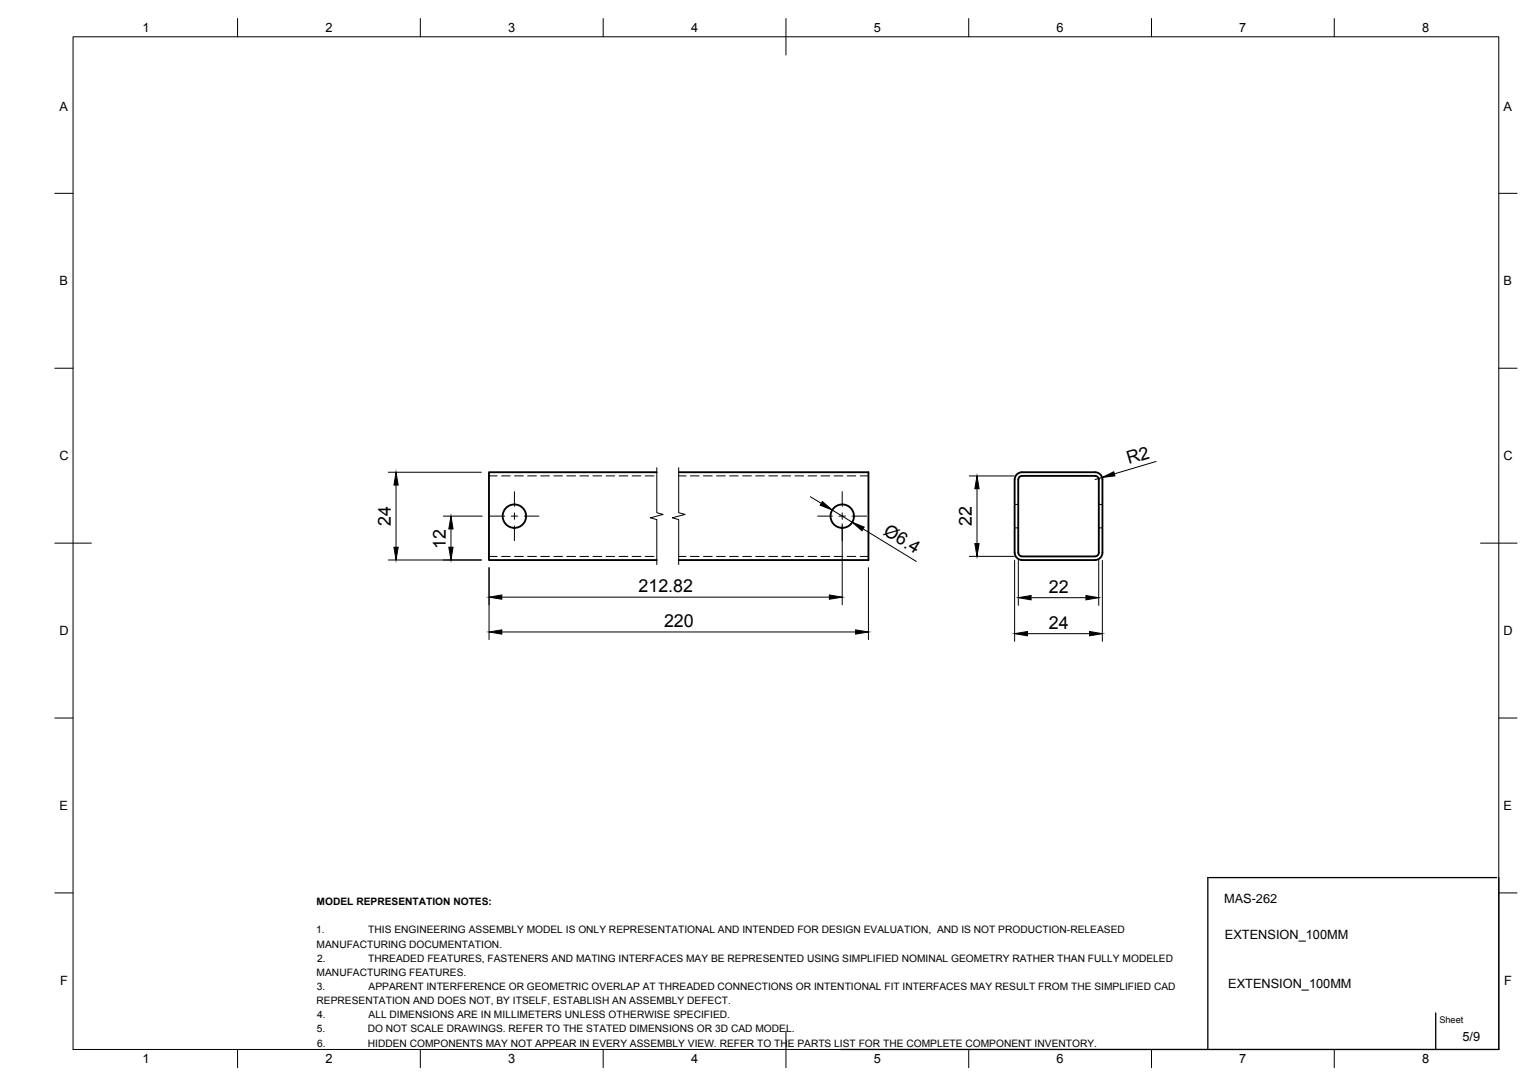
ISO-10303-21;
HEADER;
/* Generated by software containing ST-Developer
 * from STEP Tools, Inc. (www.steptools.com) 
 */

FILE_DESCRIPTION(
/* description */ (''),
/* implementation_level */ '2;1');

FILE_NAME(
/* name */ 'EXTENSION_100MM.step',
/* time_stamp */ '2026-10-07T02:13:48+06:00',
/* author */ (''),
/* organization */ (''),
/* preprocessor_version */ 'ST-DEVELOPER v20.2',
/* originating_system */ 'Autodesk Translation Framework v15.15.0.0',
/* authorisation */ '');

FILE_SCHEMA (('AUTOMOTIVE_DESIGN { 1 0 10303 214 3 1 1 }'));
ENDSEC;

DATA;
#10=MECHANICAL_DESIGN_GEOMETRIC_PRESENTATION_REPRESENTATION('',(#116),#17042);
#92=SHAPE_REPRESENTATION_RELATIONSHIP('SRR','None',#17088,#104);
#104=ADVANCED_BREP_SHAPE_REPRESENTATION('',(#128),#17032);
#116=STYLED_ITEM('',(#17154),#128);
#128=MANIFOLD_SOLID_BREP('Body1',#8117);
#148=FACE_BOUND('',#1141,.T.);
#149=FACE_BOUND('',#1145,.T.);
#150=FACE_BOUND('',#1146,.T.);
#151=FACE_BOUND('',#1151,.T.);
#152=FACE_BOUND('',#1152,.T.);
#153=FACE_BOUND('',#1157,.T.);
#154=FACE_BOUND('',#1158,.T.);
#155=FACE_BOUND('',#1163,.T.);
#156=FACE_BOUND('',#1164,.T.);
#157=FACE_BOUND('',#1167,.T.);
#360=PLANE('',#8614);
#361=PLANE('',#8623);
#362=PLANE('',#8626);
#363=PLANE('',#8629);
#364=PLANE('',#8632);
#365=PLANE('',#8635);
#366=PLANE('',#8638);
#367=PLANE('',#8641);
#368=PLANE('',#8644);
#369=PLANE('',#8647);
#649=FACE_OUTER_BOUND('',#1136,.T.);
#650=FACE_OUTER_BOUND('',#1137,.T.);
#651=FACE_OUTER_BOUND('',#1138,.T.);
#652=FACE_OUTER_BOUND('',#1139,.T.);
#653=FACE_OUTER_BOUND('',#1140,.T.);
#654=FACE_OUTER_BOUND('',#1142,.T.);
#655=FACE_OUTER_BOUND('',#1143,.T.);
#656=FACE_OUTER_BOUND('',#1144,.T.);
#657=FACE_OUTER_BOUND('',#1147,.T.);
#658=FACE_OUTER_BOUND('',#1148,.T.);
#659=FACE_OUTER_BOUND('',#1149,.T.);
#660=FACE_OUTER_BOUND('',#1150,.T.);
#661=FACE_OUTER_BOUND('',#1153,.T.);
#662=FACE_OUTER_BOUND('',#1154,.T.);
#663=FACE_OUTER_BOUND('',#1155,.T.);
#664=FACE_OUTER_BOUND('',#1156,.T.);
#665=FACE_OUTER_BOUND('',#1159,.T.);
#666=FACE_OUTER_BOUND('',#1160,.T.);
#667=FACE_OUTER_BOUND('',#1161,.T.);
#668=FACE_OUTER_BOUND('',#1162,.T.);
#669=FACE_OUTER_BOUND('',#1165,.T.);
#670=FACE_OUTER_BOUND('',#1166,.T.);
#1136=EDGE_LOOP('',(#6001,#6002,#6003,#6004));
#1137=EDGE_LOOP('',(#6005,#6006,#6007,#6008));
#1138=EDGE_LOOP('',(#6009,#6010,#6011,#6012));
#1139=EDGE_LOOP('',(#6013,#6014,#6015,#6016));
#1140=EDGE_LOOP('',(#6017,#6018,#6019,#6020,#6021,#6022,#6023,#6024));
#1141=EDGE_LOOP('',(#6025,#6026,#6027,#6028,#6029,#6030,#6031,#6032));
#1142=EDGE_LOOP('',(#6033,#6034,#6035,#6036));
#1143=EDGE_LOOP('',(#6037,#6038,#6039,#6040));
#1144=EDGE_LOOP('',(#6041,#6042,#6043,#6044));
#1145=EDGE_LOOP('',(#6045));
#1146=EDGE_LOOP('',(#6046));
#1147=EDGE_LOOP('',(#6047,#6048,#6049,#6050));
#1148=EDGE_LOOP('',(#6051,#6052,#6053,#6054));
#1149=EDGE_LOOP('',(#6055,#6056,#6057,#6058));
#1150=EDGE_LOOP('',(#6059,#6060,#6061,#6062));
#1151=EDGE_LOOP('',(#6063));
#1152=EDGE_LOOP('',(#6064));
#1153=EDGE_LOOP('',(#6065,#6066,#6067,#6068));
#1154=EDGE_LOOP('',(#6069,#6070,#6071,#6072));
#1155=EDGE_LOOP('',(#6073,#6074,#6075,#6076));
#1156=EDGE_LOOP('',(#6077,#6078,#6079,#6080));
#1157=EDGE_LOOP('',(#6081));
#1158=EDGE_LOOP('',(#6082));
#1159=EDGE_LOOP('',(#6083,#6084,#6085,#6086));
#1160=EDGE_LOOP('',(#6087,#6088,#6089,#6090));
#1161=EDGE_LOOP('',(#6091,#6092,#6093,#6094));
#1162=EDGE_LOOP('',(#6095,#6096,#6097,#6098));
#1163=EDGE_LOOP('',(#6099));
#1164=EDGE_LOOP('',(#6100));
#1165=EDGE_LOOP('',(#6101,#6102,#6103,#6104));
#1166=EDGE_LOOP('',(#6105,#6106,#6107,#6108,#6109,#6110,#6111,#6112));
#1167=EDGE_LOOP('',(#6113,#6114,#6115,#6116,#6117,#6118,#6119,#6120));
#1642=CIRCLE('',#8603,3.20000000000001);
#1643=CIRCLE('',#8604,3.20000000000001);
#1644=CIRCLE('',#8606,3.20000000000001);
#1645=CIRCLE('',#8607,3.20000000000001);
#1646=CIRCLE('',#8609,3.2);
#1647=CIRCLE('',#8610,3.2);
#1648=CIRCLE('',#8612,3.2);
#1649=CIRCLE('',#8613,3.2);
#1650=CIRCLE('',#8615,2.);
#1651=CIRCLE('',#8616,2.);
#1652=CIRCLE('',#8617,2.);
#1653=CIRCLE('',#8618,2.);
#1654=CIRCLE('',#8619,0.999999999999999);
#1655=CIRCLE('',#8620,0.999999999999999);
#1656=CIRCLE('',#8621,0.999999999999999);
#1657=CIRCLE('',#8622,1.);
#1658=CIRCLE('',#8625,0.999999999999999);
#1659=CIRCLE('',#8628,0.999999999999999);
#1660=CIRCLE('',#8631,1.);
#1661=CIRCLE('',#8634,0.999999999999999);
#1662=CIRCLE('',#8637,2.);
#1663=CIRCLE('',#8640,2.);
#1664=CIRCLE('',#8643,2.);
#1665=CIRCLE('',#8646,2.);
#2301=LINE('',#12839,#2879);
#2302=LINE('',#12845,#2880);
#2303=LINE('',#12851,#2881);
#2304=LINE('',#12857,#2882);
#2305=LINE('',#12864,#2883);
#2306=LINE('',#12868,#2884);
#2307=LINE('',#12872,#2885);
#2308=LINE('',#12875,#2886);
#2309=LINE('',#12880,#2887);
#2310=LINE('',#12884,#2888);
#2311=LINE('',#12888,#2889);
#2312=LINE('',#12891,#2890);
#2313=LINE('',#12894,#2891);
#2314=LINE('',#12896,#2892);
#2315=LINE('',#12897,#2893);
#2316=LINE('',#12901,#2894);
#2317=LINE('',#12904,#2895);
#2318=LINE('',#12905,#2896);
#2319=LINE('',#12909,#2897);
#2320=LINE('',#12912,#2898);
#2321=LINE('',#12913,#2899);
#2322=LINE('',#12917,#2900);
#2323=LINE('',#12920,#2901);
#2324=LINE('',#12921,#2902);
#2325=LINE('',#12926,#2903);
#2326=LINE('',#12928,#2904);
#2327=LINE('',#12929,#2905);
#2328=LINE('',#12933,#2906);
#2329=LINE('',#12936,#2907);
#2330=LINE('',#12937,#2908);
#2331=LINE('',#12941,#2909);
#2332=LINE('',#12944,#2910);
#2333=LINE('',#12945,#2911);
#2334=LINE('',#12949,#2912);
#2335=LINE('',#12952,#2913);
#2336=LINE('',#12953,#2914);
#2879=VECTOR('',#10218,3.20000000000001);
#2880=VECTOR('',#10225,3.20000000000001);
#2881=VECTOR('',#10232,3.2);
#2882=VECTOR('',#10239,3.2);
#2883=VECTOR('',#10246,20.);
#2884=VECTOR('',#10249,20.);
#2885=VECTOR('',#10252,20.);
#2886=VECTOR('',#10255,20.);
#2887=VECTOR('',#10258,20.);
#2888=VECTOR('',#10261,20.);
#2889=VECTOR('',#10264,20.);
#2890=VECTOR('',#10267,20.);
#2891=VECTOR('',#10270,20.);
#2892=VECTOR('',#10271,20.);
#2893=VECTOR('',#10272,20.);
#2894=VECTOR('',#10277,20.);
#2895=VECTOR('',#10280,20.);
#2896=VECTOR('',#10281,20.);
#2897=VECTOR('',#10286,20.);
#2898=VECTOR('',#10289,20.);
#2899=VECTOR('',#10290,20.);
#2900=VECTOR('',#10295,20.);
#2901=VECTOR('',#10298,20.);
#2902=VECTOR('',#10299,20.);
#2903=VECTOR('',#10306,20.);
#2904=VECTOR('',#10307,20.);
#2905=VECTOR('',#10308,20.);
#2906=VECTOR('',#10313,20.);
#2907=VECTOR('',#10316,20.);
#2908=VECTOR('',#10317,20.);
#2909=VECTOR('',#10322,20.);
#2910=VECTOR('',#10325,20.);
#2911=VECTOR('',#10326,20.);
#2912=VECTOR('',#10331,20.);
#2913=VECTOR('',#10334,20.);
#2914=VECTOR('',#10335,20.);
#3465=VERTEX_POINT('',#12836);
#3466=VERTEX_POINT('',#12838);
#3467=VERTEX_POINT('',#12842);
#3468=VERTEX_POINT('',#12844);
#3469=VERTEX_POINT('',#12848);
#3470=VERTEX_POINT('',#12850);
#3471=VERTEX_POINT('',#12854);
#3472=VERTEX_POINT('',#12856);
#3473=VERTEX_POINT('',#12860);
#3474=VERTEX_POINT('',#12861);
#3475=VERTEX_POINT('',#12863);
#3476=VERTEX_POINT('',#12865);
#3477=VERTEX_POINT('',#12867);
#3478=VERTEX_POINT('',#12869);
#3479=VERTEX_POINT('',#12871);
#3480=VERTEX_POINT('',#12873);
#3481=VERTEX_POINT('',#12876);
#3482=VERTEX_POINT('',#12877);
#3483=VERTEX_POINT('',#12879);
#3484=VERTEX_POINT('',#12881);
#3485=VERTEX_POINT('',#12883);
#3486=VERTEX_POINT('',#12885);
#3487=VERTEX_POINT('',#12887);
#3488=VERTEX_POINT('',#12889);
#3489=VERTEX_POINT('',#12893);
#3490=VERTEX_POINT('',#12895);
#3491=VERTEX_POINT('',#12899);
#3492=VERTEX_POINT('',#12903);
#3493=VERTEX_POINT('',#12907);
#3494=VERTEX_POINT('',#12911);
#3495=VERTEX_POINT('',#12915);
#3496=VERTEX_POINT('',#12919);
#3497=VERTEX_POINT('',#12925);
#3498=VERTEX_POINT('',#12927);
#3499=VERTEX_POINT('',#12931);
#3500=VERTEX_POINT('',#12935);
#3501=VERTEX_POINT('',#12939);
#3502=VERTEX_POINT('',#12943);
#3503=VERTEX_POINT('',#12947);
#3504=VERTEX_POINT('',#12951);
#4368=EDGE_CURVE('',#3465,#3465,#1642,.T.);
#4369=EDGE_CURVE('',#3465,#3466,#2301,.T.);
#4370=EDGE_CURVE('',#3466,#3466,#1643,.T.);
#4371=EDGE_CURVE('',#3467,#3467,#1644,.T.);
#4372=EDGE_CURVE('',#3467,#3468,#2302,.T.);
#4373=EDGE_CURVE('',#3468,#3468,#1645,.T.);
#4374=EDGE_CURVE('',#3469,#3469,#1646,.T.);
#4375=EDGE_CURVE('',#3469,#3470,#2303,.T.);
#4376=EDGE_CURVE('',#3470,#3470,#1647,.T.);
#4377=EDGE_CURVE('',#3471,#3471,#1648,.T.);
#4378=EDGE_CURVE('',#3471,#3472,#2304,.T.);
#4379=EDGE_CURVE('',#3472,#3472,#1649,.T.);
#4380=EDGE_CURVE('',#3473,#3474,#1650,.T.);
#4381=EDGE_CURVE('',#3474,#3475,#2305,.T.);
#4382=EDGE_CURVE('',#3475,#3476,#1651,.T.);
#4383=EDGE_CURVE('',#3476,#3477,#2306,.T.);
#4384=EDGE_CURVE('',#3477,#3478,#1652,.T.);
#4385=EDGE_CURVE('',#3478,#3479,#2307,.T.);
#4386=EDGE_CURVE('',#3479,#3480,#1653,.T.);
#4387=EDGE_CURVE('',#3480,#3473,#2308,.T.);
#4388=EDGE_CURVE('',#3481,#3482,#1654,.T.);
#4389=EDGE_CURVE('',#3482,#3483,#2309,.T.);
#4390=EDGE_CURVE('',#3483,#3484,#1655,.T.);
#4391=EDGE_CURVE('',#3484,#3485,#2310,.T.);
#4392=EDGE_CURVE('',#3485,#3486,#1656,.T.);
#4393=EDGE_CURVE('',#3486,#3487,#2311,.T.);
#4394=EDGE_CURVE('',#3487,#3488,#1657,.T.);
#4395=EDGE_CURVE('',#3488,#3481,#2312,.T.);
#4396=EDGE_CURVE('',#3489,#3482,#2313,.T.);
#4397=EDGE_CURVE('',#3490,#3489,#2314,.T.);
#4398=EDGE_CURVE('',#3483,#3490,#2315,.T.);
#4399=EDGE_CURVE('',#3491,#3490,#1658,.T.);
#4400=EDGE_CURVE('',#3484,#3491,#2316,.T.);
#4401=EDGE_CURVE('',#3492,#3491,#2317,.T.);
#4402=EDGE_CURVE('',#3485,#3492,#2318,.T.);
#4403=EDGE_CURVE('',#3493,#3492,#1659,.T.);
#4404=EDGE_CURVE('',#3486,#3493,#2319,.T.);
#4405=EDGE_CURVE('',#3494,#3493,#2320,.T.);
#4406=EDGE_CURVE('',#3487,#3494,#2321,.T.);
#4407=EDGE_CURVE('',#3495,#3494,#1660,.T.);
#4408=EDGE_CURVE('',#3488,#3495,#2322,.T.);
#4409=EDGE_CURVE('',#3496,#3495,#2323,.T.);
#4410=EDGE_CURVE('',#3481,#3496,#2324,.T.);
#4411=EDGE_CURVE('',#3489,#3496,#1661,.T.);
#4412=EDGE_CURVE('',#3497,#3474,#2325,.T.);
#4413=EDGE_CURVE('',#3498,#3497,#2326,.T.);
#4414=EDGE_CURVE('',#3475,#3498,#2327,.T.);
#4415=EDGE_CURVE('',#3499,#3498,#1662,.T.);
#4416=EDGE_CURVE('',#3476,#3499,#2328,.T.);
#4417=EDGE_CURVE('',#3500,#3499,#2329,.T.);
#4418=EDGE_CURVE('',#3477,#3500,#2330,.T.);
#4419=EDGE_CURVE('',#3501,#3500,#1663,.T.);
#4420=EDGE_CURVE('',#3478,#3501,#2331,.T.);
#4421=EDGE_CURVE('',#3502,#3501,#2332,.T.);
#4422=EDGE_CURVE('',#3479,#3502,#2333,.T.);
#4423=EDGE_CURVE('',#3503,#3502,#1664,.T.);
#4424=EDGE_CURVE('',#3480,#3503,#2334,.T.);
#4425=EDGE_CURVE('',#3504,#3503,#2335,.T.);
#4426=EDGE_CURVE('',#3473,#3504,#2336,.T.);
#4427=EDGE_CURVE('',#3497,#3504,#1665,.T.);
#6001=ORIENTED_EDGE('',*,*,#4368,.F.);
#6002=ORIENTED_EDGE('',*,*,#4369,.T.);
#6003=ORIENTED_EDGE('',*,*,#4370,.F.);
#6004=ORIENTED_EDGE('',*,*,#4369,.F.);
#6005=ORIENTED_EDGE('',*,*,#4371,.F.);
#6006=ORIENTED_EDGE('',*,*,#4372,.T.);
#6007=ORIENTED_EDGE('',*,*,#4373,.F.);
#6008=ORIENTED_EDGE('',*,*,#4372,.F.);
#6009=ORIENTED_EDGE('',*,*,#4374,.F.);
#6010=ORIENTED_EDGE('',*,*,#4375,.T.);
#6011=ORIENTED_EDGE('',*,*,#4376,.F.);
#6012=ORIENTED_EDGE('',*,*,#4375,.F.);
#6013=ORIENTED_EDGE('',*,*,#4377,.F.);
#6014=ORIENTED_EDGE('',*,*,#4378,.T.);
#6015=ORIENTED_EDGE('',*,*,#4379,.F.);
#6016=ORIENTED_EDGE('',*,*,#4378,.F.);
#6017=ORIENTED_EDGE('',*,*,#4380,.T.);
#6018=ORIENTED_EDGE('',*,*,#4381,.T.);
#6019=ORIENTED_EDGE('',*,*,#4382,.T.);
#6020=ORIENTED_EDGE('',*,*,#4383,.T.);
#6021=ORIENTED_EDGE('',*,*,#4384,.T.);
#6022=ORIENTED_EDGE('',*,*,#4385,.T.);
#6023=ORIENTED_EDGE('',*,*,#4386,.T.);
#6024=ORIENTED_EDGE('',*,*,#4387,.T.);
#6025=ORIENTED_EDGE('',*,*,#4388,.T.);
#6026=ORIENTED_EDGE('',*,*,#4389,.T.);
#6027=ORIENTED_EDGE('',*,*,#4390,.T.);
#6028=ORIENTED_EDGE('',*,*,#4391,.T.);
#6029=ORIENTED_EDGE('',*,*,#4392,.T.);
#6030=ORIENTED_EDGE('',*,*,#4393,.T.);
#6031=ORIENTED_EDGE('',*,*,#4394,.T.);
#6032=ORIENTED_EDGE('',*,*,#4395,.T.);
#6033=ORIENTED_EDGE('',*,*,#4396,.F.);
#6034=ORIENTED_EDGE('',*,*,#4397,.F.);
#6035=ORIENTED_EDGE('',*,*,#4398,.F.);
#6036=ORIENTED_EDGE('',*,*,#4389,.F.);
#6037=ORIENTED_EDGE('',*,*,#4398,.T.);
#6038=ORIENTED_EDGE('',*,*,#4399,.F.);
#6039=ORIENTED_EDGE('',*,*,#4400,.F.);
#6040=ORIENTED_EDGE('',*,*,#4390,.F.);
#6041=ORIENTED_EDGE('',*,*,#4400,.T.);
#6042=ORIENTED_EDGE('',*,*,#4401,.F.);
#6043=ORIENTED_EDGE('',*,*,#4402,.F.);
#6044=ORIENTED_EDGE('',*,*,#4391,.F.);
#6045=ORIENTED_EDGE('',*,*,#4373,.T.);
#6046=ORIENTED_EDGE('',*,*,#4379,.T.);
#6047=ORIENTED_EDGE('',*,*,#4402,.T.);
#6048=ORIENTED_EDGE('',*,*,#4403,.F.);
#6049=ORIENTED_EDGE('',*,*,#4404,.F.);
#6050=ORIENTED_EDGE('',*,*,#4392,.F.);
#6051=ORIENTED_EDGE('',*,*,#4404,.T.);
#6052=ORIENTED_EDGE('',*,*,#4405,.F.);
#6053=ORIENTED_EDGE('',*,*,#4406,.F.);
#6054=ORIENTED_EDGE('',*,*,#4393,.F.);
#6055=ORIENTED_EDGE('',*,*,#4406,.T.);
#6056=ORIENTED_EDGE('',*,*,#4407,.F.);
#6057=ORIENTED_EDGE('',*,*,#4408,.F.);
#6058=ORIENTED_EDGE('',*,*,#4394,.F.);
#6059=ORIENTED_EDGE('',*,*,#4408,.T.);
#6060=ORIENTED_EDGE('',*,*,#4409,.F.);
#6061=ORIENTED_EDGE('',*,*,#4410,.F.);
#6062=ORIENTED_EDGE('',*,*,#4395,.F.);
#6063=ORIENTED_EDGE('',*,*,#4368,.T.);
#6064=ORIENTED_EDGE('',*,*,#4374,.T.);
#6065=ORIENTED_EDGE('',*,*,#4410,.T.);
#6066=ORIENTED_EDGE('',*,*,#4411,.F.);
#6067=ORIENTED_EDGE('',*,*,#4396,.T.);
#6068=ORIENTED_EDGE('',*,*,#4388,.F.);
#6069=ORIENTED_EDGE('',*,*,#4412,.F.);
#6070=ORIENTED_EDGE('',*,*,#4413,.F.);
#6071=ORIENTED_EDGE('',*,*,#4414,.F.);
#6072=ORIENTED_EDGE('',*,*,#4381,.F.);
#6073=ORIENTED_EDGE('',*,*,#4414,.T.);
#6074=ORIENTED_EDGE('',*,*,#4415,.F.);
#6075=ORIENTED_EDGE('',*,*,#4416,.F.);
#6076=ORIENTED_EDGE('',*,*,#4382,.F.);
#6077=ORIENTED_EDGE('',*,*,#4416,.T.);
#6078=ORIENTED_EDGE('',*,*,#4417,.F.);
#6079=ORIENTED_EDGE('',*,*,#4418,.F.);
#6080=ORIENTED_EDGE('',*,*,#4383,.F.);
#6081=ORIENTED_EDGE('',*,*,#4370,.T.);
#6082=ORIENTED_EDGE('',*,*,#4376,.T.);
#6083=ORIENTED_EDGE('',*,*,#4418,.T.);
#6084=ORIENTED_EDGE('',*,*,#4419,.F.);
#6085=ORIENTED_EDGE('',*,*,#4420,.F.);
#6086=ORIENTED_EDGE('',*,*,#4384,.F.);
#6087=ORIENTED_EDGE('',*,*,#4420,.T.);
#6088=ORIENTED_EDGE('',*,*,#4421,.F.);
#6089=ORIENTED_EDGE('',*,*,#4422,.F.);
#6090=ORIENTED_EDGE('',*,*,#4385,.F.);
#6091=ORIENTED_EDGE('',*,*,#4422,.T.);
#6092=ORIENTED_EDGE('',*,*,#4423,.F.);
#6093=ORIENTED_EDGE('',*,*,#4424,.F.);
#6094=ORIENTED_EDGE('',*,*,#4386,.F.);
#6095=ORIENTED_EDGE('',*,*,#4424,.T.);
#6096=ORIENTED_EDGE('',*,*,#4425,.F.);
#6097=ORIENTED_EDGE('',*,*,#4426,.F.);
#6098=ORIENTED_EDGE('',*,*,#4387,.F.);
#6099=ORIENTED_EDGE('',*,*,#4371,.T.);
#6100=ORIENTED_EDGE('',*,*,#4377,.T.);
#6101=ORIENTED_EDGE('',*,*,#4426,.T.);
#6102=ORIENTED_EDGE('',*,*,#4427,.F.);
#6103=ORIENTED_EDGE('',*,*,#4412,.T.);
#6104=ORIENTED_EDGE('',*,*,#4380,.F.);
#6105=ORIENTED_EDGE('',*,*,#4427,.T.);
#6106=ORIENTED_EDGE('',*,*,#4425,.T.);
#6107=ORIENTED_EDGE('',*,*,#4423,.T.);
#6108=ORIENTED_EDGE('',*,*,#4421,.T.);
#6109=ORIENTED_EDGE('',*,*,#4419,.T.);
#6110=ORIENTED_EDGE('',*,*,#4417,.T.);
#6111=ORIENTED_EDGE('',*,*,#4415,.T.);
#6112=ORIENTED_EDGE('',*,*,#4413,.T.);
#6113=ORIENTED_EDGE('',*,*,#4411,.T.);
#6114=ORIENTED_EDGE('',*,*,#4409,.T.);
#6115=ORIENTED_EDGE('',*,*,#4407,.T.);
#6116=ORIENTED_EDGE('',*,*,#4405,.T.);
#6117=ORIENTED_EDGE('',*,*,#4403,.T.);
#6118=ORIENTED_EDGE('',*,*,#4401,.T.);
#6119=ORIENTED_EDGE('',*,*,#4399,.T.);
#6120=ORIENTED_EDGE('',*,*,#4397,.T.);
#7518=CYLINDRICAL_SURFACE('',#8602,3.20000000000001);
#7519=CYLINDRICAL_SURFACE('',#8605,3.20000000000001);
#7520=CYLINDRICAL_SURFACE('',#8608,3.2);
#7521=CYLINDRICAL_SURFACE('',#8611,3.2);
#7522=CYLINDRICAL_SURFACE('',#8624,0.999999999999999);
#7523=CYLINDRICAL_SURFACE('',#8627,0.999999999999999);
#7524=CYLINDRICAL_SURFACE('',#8630,1.);
#7525=CYLINDRICAL_SURFACE('',#8633,0.999999999999999);
#7526=CYLINDRICAL_SURFACE('',#8636,2.);
#7527=CYLINDRICAL_SURFACE('',#8639,2.);
#7528=CYLINDRICAL_SURFACE('',#8642,2.);
#7529=CYLINDRICAL_SURFACE('',#8645,2.);
#7811=ADVANCED_FACE('',(#649),#7518,.F.);
#7812=ADVANCED_FACE('',(#650),#7519,.F.);
#7813=ADVANCED_FACE('',(#651),#7520,.F.);
#7814=ADVANCED_FACE('',(#652),#7521,.F.);
#7815=ADVANCED_FACE('',(#653,#148),#360,.F.);
#7816=ADVANCED_FACE('',(#654),#361,.T.);
#7817=ADVANCED_FACE('',(#655),#7522,.F.);
#7818=ADVANCED_FACE('',(#656,#149,#150),#362,.T.);
#7819=ADVANCED_FACE('',(#657),#7523,.F.);
#7820=ADVANCED_FACE('',(#658),#363,.T.);
#7821=ADVANCED_FACE('',(#659),#7524,.F.);
#7822=ADVANCED_FACE('',(#660,#151,#152),#364,.T.);
#7823=ADVANCED_FACE('',(#661),#7525,.F.);
#7824=ADVANCED_FACE('',(#662),#365,.T.);
#7825=ADVANCED_FACE('',(#663),#7526,.T.);
#7826=ADVANCED_FACE('',(#664,#153,#154),#366,.T.);
#7827=ADVANCED_FACE('',(#665),#7527,.T.);
#7828=ADVANCED_FACE('',(#666),#367,.T.);
#7829=ADVANCED_FACE('',(#667),#7528,.T.);
#7830=ADVANCED_FACE('',(#668,#155,#156),#368,.T.);
#7831=ADVANCED_FACE('',(#669),#7529,.T.);
#7832=ADVANCED_FACE('',(#670,#157),#369,.T.);
#8117=CLOSED_SHELL('',(#7811,#7812,#7813,#7814,#7815,#7816,#7817,#7818,
#7819,#7820,#7821,#7822,#7823,#7824,#7825,#7826,#7827,#7828,#7829,#7830,
#7831,#7832));
#8601=AXIS2_PLACEMENT_3D('',#12834,#10212,#10213);
#8602=AXIS2_PLACEMENT_3D('',#12835,#10214,#10215);
#8603=AXIS2_PLACEMENT_3D('',#12837,#10216,#10217);
#8604=AXIS2_PLACEMENT_3D('',#12840,#10219,#10220);
#8605=AXIS2_PLACEMENT_3D('',#12841,#10221,#10222);
#8606=AXIS2_PLACEMENT_3D('',#12843,#10223,#10224);
#8607=AXIS2_PLACEMENT_3D('',#12846,#10226,#10227);
#8608=AXIS2_PLACEMENT_3D('',#12847,#10228,#10229);
#8609=AXIS2_PLACEMENT_3D('',#12849,#10230,#10231);
#8610=AXIS2_PLACEMENT_3D('',#12852,#10233,#10234);
#8611=AXIS2_PLACEMENT_3D('',#12853,#10235,#10236);
#8612=AXIS2_PLACEMENT_3D('',#12855,#10237,#10238);
#8613=AXIS2_PLACEMENT_3D('',#12858,#10240,#10241);
#8614=AXIS2_PLACEMENT_3D('',#12859,#10242,#10243);
#8615=AXIS2_PLACEMENT_3D('',#12862,#10244,#10245);
#8616=AXIS2_PLACEMENT_3D('',#12866,#10247,#10248);
#8617=AXIS2_PLACEMENT_3D('',#12870,#10250,#10251);
#8618=AXIS2_PLACEMENT_3D('',#12874,#10253,#10254);
#8619=AXIS2_PLACEMENT_3D('',#12878,#10256,#10257);
#8620=AXIS2_PLACEMENT_3D('',#12882,#10259,#10260);
#8621=AXIS2_PLACEMENT_3D('',#12886,#10262,#10263);
#8622=AXIS2_PLACEMENT_3D('',#12890,#10265,#10266);
#8623=AXIS2_PLACEMENT_3D('',#12892,#10268,#10269);
#8624=AXIS2_PLACEMENT_3D('',#12898,#10273,#10274);
#8625=AXIS2_PLACEMENT_3D('',#12900,#10275,#10276);
#8626=AXIS2_PLACEMENT_3D('',#12902,#10278,#10279);
#8627=AXIS2_PLACEMENT_3D('',#12906,#10282,#10283);
#8628=AXIS2_PLACEMENT_3D('',#12908,#10284,#10285);
#8629=AXIS2_PLACEMENT_3D('',#12910,#10287,#10288);
#8630=AXIS2_PLACEMENT_3D('',#12914,#10291,#10292);
#8631=AXIS2_PLACEMENT_3D('',#12916,#10293,#10294);
#8632=AXIS2_PLACEMENT_3D('',#12918,#10296,#10297);
#8633=AXIS2_PLACEMENT_3D('',#12922,#10300,#10301);
#8634=AXIS2_PLACEMENT_3D('',#12923,#10302,#10303);
#8635=AXIS2_PLACEMENT_3D('',#12924,#10304,#10305);
#8636=AXIS2_PLACEMENT_3D('',#12930,#10309,#10310);
#8637=AXIS2_PLACEMENT_3D('',#12932,#10311,#10312);
#8638=AXIS2_PLACEMENT_3D('',#12934,#10314,#10315);
#8639=AXIS2_PLACEMENT_3D('',#12938,#10318,#10319);
#8640=AXIS2_PLACEMENT_3D('',#12940,#10320,#10321);
#8641=AXIS2_PLACEMENT_3D('',#12942,#10323,#10324);
#8642=AXIS2_PLACEMENT_3D('',#12946,#10327,#10328);
#8643=AXIS2_PLACEMENT_3D('',#12948,#10329,#10330);
#8644=AXIS2_PLACEMENT_3D('',#12950,#10332,#10333);
#8645=AXIS2_PLACEMENT_3D('',#12954,#10336,#10337);
#8646=AXIS2_PLACEMENT_3D('',#12955,#10338,#10339);
#8647=AXIS2_PLACEMENT_3D('',#12956,#10340,#10341);
#10212=DIRECTION('axis',(0.,0.,1.));
#10213=DIRECTION('refdir',(1.,0.,0.));
#10214=DIRECTION('center_axis',(1.,0.,0.));
#10215=DIRECTION('ref_axis',(0.,1.,0.));
#10216=DIRECTION('center_axis',(1.,0.,0.));
#10217=DIRECTION('ref_axis',(0.,1.,0.));
#10218=DIRECTION('',(1.,0.,0.));
#10219=DIRECTION('center_axis',(-1.,0.,0.));
#10220=DIRECTION('ref_axis',(0.,1.,0.));
#10221=DIRECTION('center_axis',(1.,0.,0.));
#10222=DIRECTION('ref_axis',(0.,1.,0.));
#10223=DIRECTION('center_axis',(1.,0.,0.));
#10224=DIRECTION('ref_axis',(0.,1.,0.));
#10225=DIRECTION('',(1.,0.,0.));
#10226=DIRECTION('center_axis',(-1.,0.,0.));
#10227=DIRECTION('ref_axis',(0.,1.,0.));
#10228=DIRECTION('center_axis',(1.,0.,0.));
#10229=DIRECTION('ref_axis',(0.,1.,0.));
#10230=DIRECTION('center_axis',(1.,0.,0.));
#10231=DIRECTION('ref_axis',(0.,1.,0.));
#10232=DIRECTION('',(1.,0.,0.));
#10233=DIRECTION('center_axis',(-1.,0.,0.));
#10234=DIRECTION('ref_axis',(0.,1.,0.));
#10235=DIRECTION('center_axis',(1.,0.,0.));
#10236=DIRECTION('ref_axis',(0.,1.,0.));
#10237=DIRECTION('center_axis',(1.,0.,0.));
#10238=DIRECTION('ref_axis',(0.,1.,0.));
#10239=DIRECTION('',(1.,0.,0.));
#10240=DIRECTION('center_axis',(-1.,0.,0.));
#10241=DIRECTION('ref_axis',(0.,1.,0.));
#10242=DIRECTION('center_axis',(0.,0.,1.));
#10243=DIRECTION('ref_axis',(1.,0.,0.));
#10244=DIRECTION('center_axis',(0.,0.,-1.));
#10245=DIRECTION('ref_axis',(1.11022302462516E-15,1.,0.));
#10246=DIRECTION('',(1.,0.,0.));
#10247=DIRECTION('center_axis',(0.,0.,-1.));
#10248=DIRECTION('ref_axis',(1.,-1.11022302462516E-15,0.));
#10249=DIRECTION('',(0.,-1.,0.));
#10250=DIRECTION('center_axis',(0.,0.,-1.));
#10251=DIRECTION('ref_axis',(0.,-1.,0.));
#10252=DIRECTION('',(-1.,1.38777878078145E-16,0.));
#10253=DIRECTION('center_axis',(0.,0.,-1.));
#10254=DIRECTION('ref_axis',(-1.,1.11022302462516E-15,0.));
#10255=DIRECTION('',(0.,1.,0.));
#10256=DIRECTION('center_axis',(0.,0.,1.));
#10257=DIRECTION('ref_axis',(1.,0.,0.));
#10258=DIRECTION('',(-1.,0.,0.));
#10259=DIRECTION('center_axis',(0.,0.,1.));
#10260=DIRECTION('ref_axis',(0.,1.,0.));
#10261=DIRECTION('',(0.,-1.,0.));
#10262=DIRECTION('center_axis',(0.,0.,1.));
#10263=DIRECTION('ref_axis',(-1.,0.,0.));
#10264=DIRECTION('',(1.,-1.38777878078145E-16,0.));
#10265=DIRECTION('center_axis',(0.,0.,1.));
#10266=DIRECTION('ref_axis',(0.,-1.,0.));
#10267=DIRECTION('',(0.,1.,0.));
#10268=DIRECTION('center_axis',(0.,-1.,0.));
#10269=DIRECTION('ref_axis',(1.,0.,0.));
#10270=DIRECTION('',(0.,0.,-1.));
#10271=DIRECTION('',(1.,0.,0.));
#10272=DIRECTION('',(0.,0.,1.));
#10273=DIRECTION('center_axis',(0.,0.,1.));
#10274=DIRECTION('ref_axis',(0.,1.,0.));
#10275=DIRECTION('center_axis',(0.,0.,-1.));
#10276=DIRECTION('ref_axis',(0.,1.,0.));
#10277=DIRECTION('',(0.,0.,1.));
#10278=DIRECTION('center_axis',(1.,0.,0.));
#10279=DIRECTION('ref_axis',(0.,1.,0.));
#10280=DIRECTION('',(0.,1.,0.));
#10281=DIRECTION('',(0.,0.,1.));
#10282=DIRECTION('center_axis',(0.,0.,1.));
#10283=DIRECTION('ref_axis',(-1.,0.,0.));
#10284=DIRECTION('center_axis',(0.,0.,-1.));
#10285=DIRECTION('ref_axis',(-1.,0.,0.));
#10286=DIRECTION('',(0.,0.,1.));
#10287=DIRECTION('center_axis',(1.38777878078145E-16,1.,0.));
#10288=DIRECTION('ref_axis',(-1.,1.38777878078145E-16,0.));
#10289=DIRECTION('',(-1.,1.38777878078145E-16,0.));
#10290=DIRECTION('',(0.,0.,1.));
#10291=DIRECTION('center_axis',(0.,0.,1.));
#10292=DIRECTION('ref_axis',(0.,-1.,0.));
#10293=DIRECTION('center_axis',(0.,0.,-1.));
#10294=DIRECTION('ref_axis',(0.,-1.,0.));
#10295=DIRECTION('',(0.,0.,1.));
#10296=DIRECTION('center_axis',(-1.,0.,0.));
#10297=DIRECTION('ref_axis',(0.,-1.,0.));
#10298=DIRECTION('',(0.,-1.,0.));
#10299=DIRECTION('',(0.,0.,1.));
#10300=DIRECTION('center_axis',(0.,0.,1.));
#10301=DIRECTION('ref_axis',(1.,0.,0.));
#10302=DIRECTION('center_axis',(0.,0.,-1.));
#10303=DIRECTION('ref_axis',(1.,0.,0.));
#10304=DIRECTION('center_axis',(0.,1.,0.));
#10305=DIRECTION('ref_axis',(-1.,0.,0.));
#10306=DIRECTION('',(0.,0.,-1.));
#10307=DIRECTION('',(-1.,0.,0.));
#10308=DIRECTION('',(0.,0.,1.));
#10309=DIRECTION('center_axis',(0.,0.,1.));
#10310=DIRECTION('ref_axis',(1.,-1.11022302462516E-15,0.));
#10311=DIRECTION('center_axis',(0.,0.,1.));
#10312=DIRECTION('ref_axis',(1.,-1.11022302462516E-15,0.));
#10313=DIRECTION('',(0.,0.,1.));
#10314=DIRECTION('center_axis',(1.,0.,0.));
#10315=DIRECTION('ref_axis',(0.,1.,0.));
#10316=DIRECTION('',(0.,1.,0.));
#10317=DIRECTION('',(0.,0.,1.));
#10318=DIRECTION('center_axis',(0.,0.,1.));
#10319=DIRECTION('ref_axis',(0.,-1.,0.));
#10320=DIRECTION('center_axis',(0.,0.,1.));
#10321=DIRECTION('ref_axis',(0.,-1.,0.));
#10322=DIRECTION('',(0.,0.,1.));
#10323=DIRECTION('center_axis',(-1.38777878078145E-16,-1.,0.));
#10324=DIRECTION('ref_axis',(1.,-1.38777878078145E-16,0.));
#10325=DIRECTION('',(1.,-1.38777878078145E-16,0.));
#10326=DIRECTION('',(0.,0.,1.));
#10327=DIRECTION('center_axis',(0.,0.,1.));
#10328=DIRECTION('ref_axis',(-1.,1.11022302462516E-15,0.));
#10329=DIRECTION('center_axis',(0.,0.,1.));
#10330=DIRECTION('ref_axis',(-1.,1.11022302462516E-15,0.));
#10331=DIRECTION('',(0.,0.,1.));
#10332=DIRECTION('center_axis',(-1.,0.,0.));
#10333=DIRECTION('ref_axis',(0.,-1.,0.));
#10334=DIRECTION('',(0.,-1.,0.));
#10335=DIRECTION('',(0.,0.,1.));
#10336=DIRECTION('center_axis',(0.,0.,1.));
#10337=DIRECTION('ref_axis',(1.11022302462516E-15,1.,0.));
#10338=DIRECTION('center_axis',(0.,0.,1.));
#10339=DIRECTION('ref_axis',(1.11022302462516E-15,1.,0.));
#10340=DIRECTION('center_axis',(0.,0.,1.));
#10341=DIRECTION('ref_axis',(1.,0.,0.));
#12834=CARTESIAN_POINT('',(0.,0.,0.));
#12835=CARTESIAN_POINT('Origin',(-6.5,6.43177298256785,249.937669285906));
#12836=CARTESIAN_POINT('',(4.5,3.23177298256785,249.937669285906));
#12837=CARTESIAN_POINT('Origin',(4.5,6.43177298256785,249.937669285906));
#12838=CARTESIAN_POINT('',(5.5,3.23177298256785,249.937669285906));
#12839=CARTESIAN_POINT('',(-6.5,3.23177298256785,249.937669285906));
#12840=CARTESIAN_POINT('Origin',(5.5,6.43177298256785,249.937669285906));
#12841=CARTESIAN_POINT('Origin',(-6.5,6.43177298256785,249.937669285906));
#12842=CARTESIAN_POINT('',(-18.5,3.23177298256785,249.937669285906));
#12843=CARTESIAN_POINT('Origin',(-18.5,6.43177298256785,249.937669285906));
#12844=CARTESIAN_POINT('',(-17.5,3.23177298256785,249.937669285906));
#12845=CARTESIAN_POINT('',(-6.5,3.23177298256785,249.937669285906));
#12846=CARTESIAN_POINT('Origin',(-17.5,6.43177298256785,249.937669285906));
#12847=CARTESIAN_POINT('Origin',(-6.5,6.43177298256785,44.0628614786648));
#12848=CARTESIAN_POINT('',(4.5,3.23177298256785,44.0628614786648));
#12849=CARTESIAN_POINT('Origin',(4.5,6.43177298256785,44.0628614786648));
#12850=CARTESIAN_POINT('',(5.5,3.23177298256785,44.0628614786648));
#12851=CARTESIAN_POINT('',(-6.5,3.23177298256785,44.0628614786648));
#12852=CARTESIAN_POINT('Origin',(5.5,6.43177298256785,44.0628614786648));
#12853=CARTESIAN_POINT('Origin',(-6.5,6.43177298256785,44.0628614786648));
#12854=CARTESIAN_POINT('',(-18.5,3.23177298256785,44.0628614786648));
#12855=CARTESIAN_POINT('Origin',(-18.5,6.43177298256785,44.0628614786648));
#12856=CARTESIAN_POINT('',(-17.5,3.23177298256785,44.0628614786648));
#12857=CARTESIAN_POINT('',(-6.5,3.23177298256785,44.0628614786648));
#12858=CARTESIAN_POINT('Origin',(-17.5,6.43177298256785,44.0628614786648));
#12859=CARTESIAN_POINT('Origin',(-6.5,6.43177298256785,36.8862095951938));
#12860=CARTESIAN_POINT('',(-18.5,16.4317729825678,36.8862095951938));
#12861=CARTESIAN_POINT('',(-16.5,18.4317729825679,36.8862095951938));
#12862=CARTESIAN_POINT('Origin',(-16.5,16.4317729825679,36.8862095951938));
#12863=CARTESIAN_POINT('',(3.5,18.4317729825679,36.8862095951938));
#12864=CARTESIAN_POINT('',(-0.499999999999999,18.4317729825679,36.8862095951938));
#12865=CARTESIAN_POINT('',(5.5,16.4317729825678,36.8862095951938));
#12866=CARTESIAN_POINT('Origin',(3.5,16.4317729825679,36.8862095951938));
#12867=CARTESIAN_POINT('',(5.5,-3.56822701743215,36.8862095951938));
#12868=CARTESIAN_POINT('',(5.5,16.4317729825678,36.8862095951938));
#12869=CARTESIAN_POINT('',(3.5,-5.56822701743215,36.8862095951938));
#12870=CARTESIAN_POINT('Origin',(3.5,-3.56822701743215,36.8862095951938));
#12871=CARTESIAN_POINT('',(-16.5,-5.56822701743215,36.8862095951938));
#12872=CARTESIAN_POINT('',(-0.499999999999999,-5.56822701743215,36.8862095951938));
#12873=CARTESIAN_POINT('',(-18.5,-3.56822701743215,36.8862095951938));
#12874=CARTESIAN_POINT('Origin',(-16.5,-3.56822701743215,36.8862095951938));
#12875=CARTESIAN_POINT('',(-18.5,-3.56822701743215,36.8862095951938));
#12876=CARTESIAN_POINT('',(4.5,16.4317729825679,36.8862095951938));
#12877=CARTESIAN_POINT('',(3.5,17.4317729825679,36.8862095951938));
#12878=CARTESIAN_POINT('Origin',(3.5,16.4317729825679,36.8862095951938));
#12879=CARTESIAN_POINT('',(-16.5,17.4317729825679,36.8862095951938));
#12880=CARTESIAN_POINT('',(-0.499999999999999,17.4317729825679,36.8862095951938));
#12881=CARTESIAN_POINT('',(-17.5,16.4317729825678,36.8862095951938));
#12882=CARTESIAN_POINT('Origin',(-16.5,16.4317729825679,36.8862095951938));
#12883=CARTESIAN_POINT('',(-17.5,-3.56822701743215,36.8862095951938));
#12884=CARTESIAN_POINT('',(-17.5,-3.56822701743215,36.8862095951938));
#12885=CARTESIAN_POINT('',(-16.5,-4.56822701743215,36.8862095951938));
#12886=CARTESIAN_POINT('Origin',(-16.5,-3.56822701743215,36.8862095951938));
#12887=CARTESIAN_POINT('',(3.5,-4.56822701743215,36.8862095951938));
#12888=CARTESIAN_POINT('',(-0.499999999999999,-4.56822701743215,36.8862095951938));
#12889=CARTESIAN_POINT('',(4.5,-3.56822701743214,36.8862095951938));
#12890=CARTESIAN_POINT('Origin',(3.5,-3.56822701743215,36.8862095951938));
#12891=CARTESIAN_POINT('',(4.5,16.4317729825679,36.8862095951938));
#12892=CARTESIAN_POINT('Origin',(-16.5,17.4317729825679,48.8862095951938));
#12893=CARTESIAN_POINT('',(3.5,17.4317729825679,256.886209595194));
#12894=CARTESIAN_POINT('',(3.5,17.4317729825679,48.8862095951938));
#12895=CARTESIAN_POINT('',(-16.5,17.4317729825679,256.886209595194));
#12896=CARTESIAN_POINT('',(-0.499999999999999,17.4317729825679,256.886209595194));
#12897=CARTESIAN_POINT('',(-16.5,17.4317729825679,48.8862095951938));
#12898=CARTESIAN_POINT('Origin',(-16.5,16.4317729825679,48.8862095951938));
#12899=CARTESIAN_POINT('',(-17.5,16.4317729825678,256.886209595194));
#12900=CARTESIAN_POINT('Origin',(-16.5,16.4317729825679,256.886209595194));
#12901=CARTESIAN_POINT('',(-17.5,16.4317729825678,48.8862095951938));
#12902=CARTESIAN_POINT('Origin',(-17.5,-3.56822701743215,48.8862095951938));
#12903=CARTESIAN_POINT('',(-17.5,-3.56822701743215,256.886209595194));
#12904=CARTESIAN_POINT('',(-17.5,-3.56822701743215,256.886209595194));
#12905=CARTESIAN_POINT('',(-17.5,-3.56822701743215,48.8862095951938));
#12906=CARTESIAN_POINT('Origin',(-16.5,-3.56822701743215,48.8862095951938));
#12907=CARTESIAN_POINT('',(-16.5,-4.56822701743215,256.886209595194));
#12908=CARTESIAN_POINT('Origin',(-16.5,-3.56822701743215,256.886209595194));
#12909=CARTESIAN_POINT('',(-16.5,-4.56822701743215,48.8862095951938));
#12910=CARTESIAN_POINT('Origin',(3.5,-4.56822701743215,48.8862095951938));
#12911=CARTESIAN_POINT('',(3.5,-4.56822701743215,256.886209595194));
#12912=CARTESIAN_POINT('',(-0.499999999999999,-4.56822701743215,256.886209595194));
#12913=CARTESIAN_POINT('',(3.5,-4.56822701743215,48.8862095951938));
#12914=CARTESIAN_POINT('Origin',(3.5,-3.56822701743215,48.8862095951938));
#12915=CARTESIAN_POINT('',(4.5,-3.56822701743214,256.886209595194));
#12916=CARTESIAN_POINT('Origin',(3.5,-3.56822701743215,256.886209595194));
#12917=CARTESIAN_POINT('',(4.5,-3.56822701743215,48.8862095951938));
#12918=CARTESIAN_POINT('Origin',(4.5,16.4317729825679,48.8862095951938));
#12919=CARTESIAN_POINT('',(4.5,16.4317729825679,256.886209595194));
#12920=CARTESIAN_POINT('',(4.5,16.4317729825679,256.886209595194));
#12921=CARTESIAN_POINT('',(4.5,16.4317729825679,48.8862095951938));
#12922=CARTESIAN_POINT('Origin',(3.5,16.4317729825679,48.8862095951938));
#12923=CARTESIAN_POINT('Origin',(3.5,16.4317729825679,256.886209595194));
#12924=CARTESIAN_POINT('Origin',(3.5,18.4317729825679,48.8862095951938));
#12925=CARTESIAN_POINT('',(-16.5,18.4317729825679,256.886209595194));
#12926=CARTESIAN_POINT('',(-16.5,18.4317729825679,48.8862095951938));
#12927=CARTESIAN_POINT('',(3.5,18.4317729825679,256.886209595194));
#12928=CARTESIAN_POINT('',(-0.499999999999999,18.4317729825679,256.886209595194));
#12929=CARTESIAN_POINT('',(3.5,18.4317729825679,48.8862095951938));
#12930=CARTESIAN_POINT('Origin',(3.5,16.4317729825679,48.8862095951938));
#12931=CARTESIAN_POINT('',(5.5,16.4317729825678,256.886209595194));
#12932=CARTESIAN_POINT('Origin',(3.5,16.4317729825679,256.886209595194));
#12933=CARTESIAN_POINT('',(5.5,16.4317729825678,48.8862095951938));
#12934=CARTESIAN_POINT('Origin',(5.5,-3.56822701743215,48.8862095951938));
#12935=CARTESIAN_POINT('',(5.5,-3.56822701743215,256.886209595194));
#12936=CARTESIAN_POINT('',(5.5,16.4317729825678,256.886209595194));
#12937=CARTESIAN_POINT('',(5.5,-3.56822701743215,48.8862095951938));
#12938=CARTESIAN_POINT('Origin',(3.5,-3.56822701743215,48.8862095951938));
#12939=CARTESIAN_POINT('',(3.5,-5.56822701743215,256.886209595194));
#12940=CARTESIAN_POINT('Origin',(3.5,-3.56822701743215,256.886209595194));
#12941=CARTESIAN_POINT('',(3.5,-5.56822701743215,48.8862095951938));
#12942=CARTESIAN_POINT('Origin',(-16.5,-5.56822701743215,48.8862095951938));
#12943=CARTESIAN_POINT('',(-16.5,-5.56822701743215,256.886209595194));
#12944=CARTESIAN_POINT('',(-0.499999999999999,-5.56822701743215,256.886209595194));
#12945=CARTESIAN_POINT('',(-16.5,-5.56822701743215,48.8862095951938));
#12946=CARTESIAN_POINT('Origin',(-16.5,-3.56822701743215,48.8862095951938));
#12947=CARTESIAN_POINT('',(-18.5,-3.56822701743215,256.886209595194));
#12948=CARTESIAN_POINT('Origin',(-16.5,-3.56822701743215,256.886209595194));
#12949=CARTESIAN_POINT('',(-18.5,-3.56822701743215,48.8862095951938));
#12950=CARTESIAN_POINT('Origin',(-18.5,16.4317729825678,48.8862095951938));
#12951=CARTESIAN_POINT('',(-18.5,16.4317729825678,256.886209595194));
#12952=CARTESIAN_POINT('',(-18.5,-3.56822701743215,256.886209595194));
#12953=CARTESIAN_POINT('',(-18.5,16.4317729825678,48.8862095951938));
#12954=CARTESIAN_POINT('Origin',(-16.5,16.4317729825679,48.8862095951938));
#12955=CARTESIAN_POINT('Origin',(-16.5,16.4317729825679,256.886209595194));
#12956=CARTESIAN_POINT('Origin',(-6.5,6.43177298256785,256.886209595194));
#17018=UNCERTAINTY_MEASURE_WITH_UNIT(LENGTH_MEASURE(0.01),#17043,
'DISTANCE_ACCURACY_VALUE',
'Maximum model space distance between geometric entities at asserted c
onnectivities');
#17028=UNCERTAINTY_MEASURE_WITH_UNIT(LENGTH_MEASURE(0.01),#17043,
'DISTANCE_ACCURACY_VALUE',
'Maximum model space distance between geometric entities at asserted c
onnectivities');
#17032=(
GEOMETRIC_REPRESENTATION_CONTEXT(3)
GLOBAL_UNCERTAINTY_ASSIGNED_CONTEXT((#17018))
GLOBAL_UNIT_ASSIGNED_CONTEXT((#17043,#17045,#17046))
REPRESENTATION_CONTEXT('','3D')
);
#17042=(
GEOMETRIC_REPRESENTATION_CONTEXT(3)
GLOBAL_UNCERTAINTY_ASSIGNED_CONTEXT((#17028))
GLOBAL_UNIT_ASSIGNED_CONTEXT((#17043,#17045,#17046))
REPRESENTATION_CONTEXT('','3D')
);
#17043=(
LENGTH_UNIT()
NAMED_UNIT(*)
SI_UNIT(.MILLI.,.METRE.)
);
#17045=(
NAMED_UNIT(*)
PLANE_ANGLE_UNIT()
SI_UNIT($,.RADIAN.)
);
#17046=(
NAMED_UNIT(*)
SI_UNIT($,.STERADIAN.)
SOLID_ANGLE_UNIT()
);
#17050=SHAPE_DEFINITION_REPRESENTATION(#17063,#17088);
#17063=PRODUCT_DEFINITION_SHAPE('',$,#17102);
#17088=SHAPE_REPRESENTATION('',(#8601),#17032);
#17098=PRODUCT_DEFINITION_CONTEXT('part definition',#17139,'design');
#17102=PRODUCT_DEFINITION('EXTENSION_100MM','EXTENSION_100MM',#17115,#17098);
#17115=PRODUCT_DEFINITION_FORMATION('',$,#17144);
#17139=APPLICATION_CONTEXT(
'Core Data for Automotive Mechanical Design Process');
#17140=PRODUCT_CONTEXT('part definition',#17139,'mechanical');
#17144=PRODUCT('EXTENSION_100MM','EXTENSION_100MM',$,(#17140));
#17154=PRESENTATION_STYLE_ASSIGNMENT((#17155));
#17155=SURFACE_STYLE_USAGE(.BOTH.,#17156);
#17156=SURFACE_SIDE_STYLE('',(#17157));
#17157=SURFACE_STYLE_FILL_AREA(#17158);
#17158=FILL_AREA_STYLE('Steel - Satin',(#17159));
#17159=FILL_AREA_STYLE_COLOUR('Steel - Satin',#17160);
#17160=COLOUR_RGB('Steel - Satin', 0.09019608, 0.27058824, 0.51372549);
ENDSEC;
END-ISO-10303-21;
